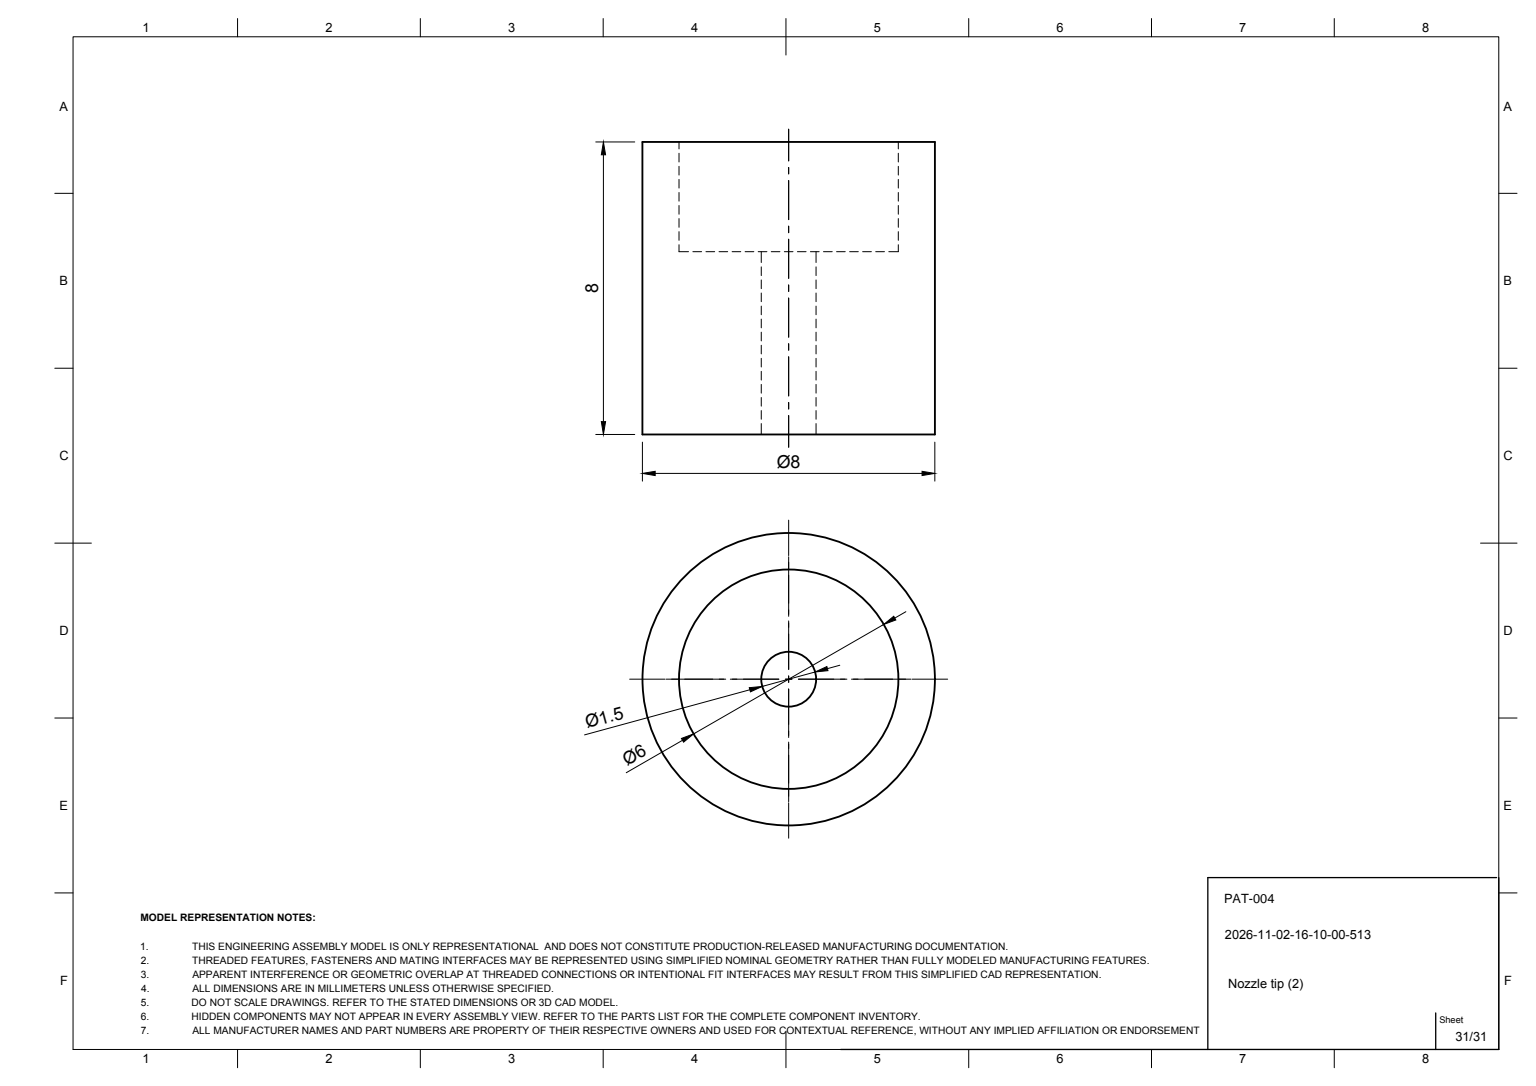
ISO-10303-21;
HEADER;
/* Generated by software containing ST-Developer
 * from STEP Tools, Inc. (www.steptools.com) 
 */

FILE_DESCRIPTION(
/* description */ ('Air blow-off nozzle station'),
/* implementation_level */ '2;1');

FILE_NAME(
/* name */ 'Nozzle tip (2).step',
/* time_stamp */ '2026-10-27T10:53:54-07:00',
/* author */ (''),
/* organization */ (''),
/* preprocessor_version */ 'ST-DEVELOPER v20.2',
/* originating_system */ 'Autodesk Translation Framework v15.17.0.0',
/* authorisation */ '');

FILE_SCHEMA (('AUTOMOTIVE_DESIGN { 1 0 10303 214 3 1 1 }'));
ENDSEC;

DATA;
#10=MECHANICAL_DESIGN_GEOMETRIC_PRESENTATION_REPRESENTATION('',(#259),#7897);
#209=SHAPE_REPRESENTATION_RELATIONSHIP('SRR','None',#8026,#234);
#234=ADVANCED_BREP_SHAPE_REPRESENTATION('',(#282),#7893);
#259=STYLED_ITEM('',(#8213),#282);
#282=MANIFOLD_SOLID_BREP('Body1',#4310);
#359=FACE_BOUND('',#1099,.T.);
#360=FACE_BOUND('',#1103,.T.);
#361=FACE_BOUND('',#1105,.T.);
#522=PLANE('',#5003);
#523=PLANE('',#5010);
#524=PLANE('',#5011);
#767=FACE_OUTER_BOUND('',#1097,.T.);
#768=FACE_OUTER_BOUND('',#1098,.T.);
#769=FACE_OUTER_BOUND('',#1100,.T.);
#770=FACE_OUTER_BOUND('',#1101,.T.);
#771=FACE_OUTER_BOUND('',#1102,.T.);
#772=FACE_OUTER_BOUND('',#1104,.T.);
#1097=EDGE_LOOP('',(#3857,#3858,#3859,#3860));
#1098=EDGE_LOOP('',(#3861));
#1099=EDGE_LOOP('',(#3862));
#1100=EDGE_LOOP('',(#3863,#3864,#3865,#3866));
#1101=EDGE_LOOP('',(#3867,#3868,#3869,#3870));
#1102=EDGE_LOOP('',(#3871));
#1103=EDGE_LOOP('',(#3872));
#1104=EDGE_LOOP('',(#3873));
#1105=EDGE_LOOP('',(#3874));
#1463=LINE('',#7703,#1817);
#1464=LINE('',#7710,#1818);
#1465=LINE('',#7716,#1819);
#1817=VECTOR('',#6223,0.3);
#1818=VECTOR('',#6232,0.0750000000000002);
#1819=VECTOR('',#6239,0.4);
#1985=CIRCLE('',#5001,0.3);
#1986=CIRCLE('',#5002,0.3);
#1987=CIRCLE('',#5004,0.0750000000000002);
#1988=CIRCLE('',#5006,0.0750000000000002);
#1989=CIRCLE('',#5008,0.4);
#1990=CIRCLE('',#5009,0.4);
#2332=VERTEX_POINT('',#7700);
#2333=VERTEX_POINT('',#7702);
#2334=VERTEX_POINT('',#7706);
#2335=VERTEX_POINT('',#7709);
#2336=VERTEX_POINT('',#7713);
#2337=VERTEX_POINT('',#7715);
#2846=EDGE_CURVE('',#2332,#2332,#1985,.T.);
#2847=EDGE_CURVE('',#2332,#2333,#1463,.T.);
#2848=EDGE_CURVE('',#2333,#2333,#1986,.T.);
#2849=EDGE_CURVE('',#2334,#2334,#1987,.T.);
#2850=EDGE_CURVE('',#2334,#2335,#1464,.T.);
#2851=EDGE_CURVE('',#2335,#2335,#1988,.T.);
#2852=EDGE_CURVE('',#2336,#2336,#1989,.T.);
#2853=EDGE_CURVE('',#2336,#2337,#1465,.T.);
#2854=EDGE_CURVE('',#2337,#2337,#1990,.T.);
#3857=ORIENTED_EDGE('',*,*,#2846,.F.);
#3858=ORIENTED_EDGE('',*,*,#2847,.T.);
#3859=ORIENTED_EDGE('',*,*,#2848,.F.);
#3860=ORIENTED_EDGE('',*,*,#2847,.F.);
#3861=ORIENTED_EDGE('',*,*,#2846,.T.);
#3862=ORIENTED_EDGE('',*,*,#2849,.F.);
#3863=ORIENTED_EDGE('',*,*,#2849,.T.);
#3864=ORIENTED_EDGE('',*,*,#2850,.T.);
#3865=ORIENTED_EDGE('',*,*,#2851,.T.);
#3866=ORIENTED_EDGE('',*,*,#2850,.F.);
#3867=ORIENTED_EDGE('',*,*,#2852,.F.);
#3868=ORIENTED_EDGE('',*,*,#2853,.T.);
#3869=ORIENTED_EDGE('',*,*,#2854,.T.);
#3870=ORIENTED_EDGE('',*,*,#2853,.F.);
#3871=ORIENTED_EDGE('',*,*,#2852,.T.);
#3872=ORIENTED_EDGE('',*,*,#2848,.T.);
#3873=ORIENTED_EDGE('',*,*,#2854,.F.);
#3874=ORIENTED_EDGE('',*,*,#2851,.F.);
#4019=CYLINDRICAL_SURFACE('',#5000,0.3);
#4020=CYLINDRICAL_SURFACE('',#5005,0.0750000000000002);
#4021=CYLINDRICAL_SURFACE('',#5007,0.4);
#4257=ADVANCED_FACE('',(#767),#4019,.F.);
#4258=ADVANCED_FACE('',(#768,#359),#522,.T.);
#4259=ADVANCED_FACE('',(#769),#4020,.F.);
#4260=ADVANCED_FACE('',(#770),#4021,.T.);
#4261=ADVANCED_FACE('',(#771,#360),#523,.T.);
#4262=ADVANCED_FACE('',(#772,#361),#524,.F.);
#4310=CLOSED_SHELL('',(#4257,#4258,#4259,#4260,#4261,#4262));
#4999=AXIS2_PLACEMENT_3D('',#7698,#6217,#6218);
#5000=AXIS2_PLACEMENT_3D('',#7699,#6219,#6220);
#5001=AXIS2_PLACEMENT_3D('',#7701,#6221,#6222);
#5002=AXIS2_PLACEMENT_3D('',#7704,#6224,#6225);
#5003=AXIS2_PLACEMENT_3D('',#7705,#6226,#6227);
#5004=AXIS2_PLACEMENT_3D('',#7707,#6228,#6229);
#5005=AXIS2_PLACEMENT_3D('',#7708,#6230,#6231);
#5006=AXIS2_PLACEMENT_3D('',#7711,#6233,#6234);
#5007=AXIS2_PLACEMENT_3D('',#7712,#6235,#6236);
#5008=AXIS2_PLACEMENT_3D('',#7714,#6237,#6238);
#5009=AXIS2_PLACEMENT_3D('',#7717,#6240,#6241);
#5010=AXIS2_PLACEMENT_3D('',#7718,#6242,#6243);
#5011=AXIS2_PLACEMENT_3D('',#7719,#6244,#6245);
#6217=DIRECTION('axis',(0.,0.,1.));
#6218=DIRECTION('refdir',(1.,0.,0.));
#6219=DIRECTION('center_axis',(0.,1.,0.));
#6220=DIRECTION('ref_axis',(1.,0.,0.));
#6221=DIRECTION('center_axis',(0.,1.,0.));
#6222=DIRECTION('ref_axis',(1.,0.,0.));
#6223=DIRECTION('',(0.,1.,0.));
#6224=DIRECTION('center_axis',(0.,-1.,0.));
#6225=DIRECTION('ref_axis',(1.,0.,0.));
#6226=DIRECTION('center_axis',(0.,1.,0.));
#6227=DIRECTION('ref_axis',(1.,0.,0.));
#6228=DIRECTION('center_axis',(0.,1.,0.));
#6229=DIRECTION('ref_axis',(1.,0.,0.));
#6230=DIRECTION('center_axis',(0.,1.,0.));
#6231=DIRECTION('ref_axis',(1.,0.,0.));
#6232=DIRECTION('',(0.,-1.,0.));
#6233=DIRECTION('center_axis',(0.,-1.,0.));
#6234=DIRECTION('ref_axis',(1.,0.,0.));
#6235=DIRECTION('center_axis',(0.,1.,0.));
#6236=DIRECTION('ref_axis',(1.,0.,0.));
#6237=DIRECTION('center_axis',(0.,1.,0.));
#6238=DIRECTION('ref_axis',(1.,0.,0.));
#6239=DIRECTION('',(0.,-1.,0.));
#6240=DIRECTION('center_axis',(0.,1.,0.));
#6241=DIRECTION('ref_axis',(1.,0.,0.));
#6242=DIRECTION('center_axis',(0.,1.,0.));
#6243=DIRECTION('ref_axis',(1.,0.,0.));
#6244=DIRECTION('center_axis',(0.,1.,0.));
#6245=DIRECTION('ref_axis',(1.,0.,0.));
#7698=CARTESIAN_POINT('',(0.,0.,0.));
#7699=CARTESIAN_POINT('Origin',(3.,-7.2,23.));
#7700=CARTESIAN_POINT('',(2.7,-7.2,23.));
#7701=CARTESIAN_POINT('Origin',(3.,-7.2,23.));
#7702=CARTESIAN_POINT('',(2.7,-6.9,23.));
#7703=CARTESIAN_POINT('',(2.7,-7.2,23.));
#7704=CARTESIAN_POINT('Origin',(3.,-6.9,23.));
#7705=CARTESIAN_POINT('Origin',(3.,-7.2,23.));
#7706=CARTESIAN_POINT('',(2.925,-7.2,23.));
#7707=CARTESIAN_POINT('Origin',(3.,-7.2,23.));
#7708=CARTESIAN_POINT('Origin',(3.,-7.7,23.));
#7709=CARTESIAN_POINT('',(2.925,-7.7,23.));
#7710=CARTESIAN_POINT('',(2.925,-7.7,23.));
#7711=CARTESIAN_POINT('Origin',(3.,-7.7,23.));
#7712=CARTESIAN_POINT('Origin',(3.,-7.7,23.));
#7713=CARTESIAN_POINT('',(2.6,-6.9,23.));
#7714=CARTESIAN_POINT('Origin',(3.,-6.9,23.));
#7715=CARTESIAN_POINT('',(2.6,-7.7,23.));
#7716=CARTESIAN_POINT('',(2.6,-7.7,23.));
#7717=CARTESIAN_POINT('Origin',(3.,-7.7,23.));
#7718=CARTESIAN_POINT('Origin',(3.,-6.9,23.));
#7719=CARTESIAN_POINT('Origin',(3.,-7.7,23.));
#7861=UNCERTAINTY_MEASURE_WITH_UNIT(LENGTH_MEASURE(0.001),#7898,
'DISTANCE_ACCURACY_VALUE',
'Maximum model space distance between geometric entities at asserted c
onnectivities');
#7865=UNCERTAINTY_MEASURE_WITH_UNIT(LENGTH_MEASURE(0.001),#7898,
'DISTANCE_ACCURACY_VALUE',
'Maximum model space distance between geometric entities at asserted c
onnectivities');
#7893=(
GEOMETRIC_REPRESENTATION_CONTEXT(3)
GLOBAL_UNCERTAINTY_ASSIGNED_CONTEXT((#7861))
GLOBAL_UNIT_ASSIGNED_CONTEXT((#7898,#7900,#7901))
REPRESENTATION_CONTEXT('','3D')
);
#7897=(
GEOMETRIC_REPRESENTATION_CONTEXT(3)
GLOBAL_UNCERTAINTY_ASSIGNED_CONTEXT((#7865))
GLOBAL_UNIT_ASSIGNED_CONTEXT((#7898,#7900,#7901))
REPRESENTATION_CONTEXT('','3D')
);
#7898=(
LENGTH_UNIT()
NAMED_UNIT(*)
SI_UNIT(.CENTI.,.METRE.)
);
#7900=(
NAMED_UNIT(*)
PLANE_ANGLE_UNIT()
SI_UNIT($,.RADIAN.)
);
#7901=(
NAMED_UNIT(*)
SI_UNIT($,.STERADIAN.)
SOLID_ANGLE_UNIT()
);
#7929=SHAPE_DEFINITION_REPRESENTATION(#7977,#8026);
#7977=PRODUCT_DEFINITION_SHAPE('',$,#8058);
#8026=SHAPE_REPRESENTATION('',(#4999),#7893);
#8030=PRODUCT_DEFINITION_CONTEXT('part definition',#8125,'design');
#8058=PRODUCT_DEFINITION('Nozzle tip (2)','Nozzle tip (2)',#8089,#8030);
#8089=PRODUCT_DEFINITION_FORMATION('',$,#8154);
#8125=APPLICATION_CONTEXT(
'Core Data for Automotive Mechanical Design Process');
#8126=PRODUCT_CONTEXT('part definition',#8125,'mechanical');
#8154=PRODUCT('Nozzle tip (2)','Nozzle tip (2)','Nozzle tip (2)',(#8126));
#8207=COLOUR_RGB('Sky Blue',0.24,0.69,0.87);
#8208=FILL_AREA_STYLE_COLOUR('',#8207);
#8209=FILL_AREA_STYLE('',(#8208));
#8210=SURFACE_STYLE_FILL_AREA(#8209);
#8211=SURFACE_SIDE_STYLE('',(#8210));
#8212=SURFACE_STYLE_USAGE(.BOTH.,#8211);
#8213=PRESENTATION_STYLE_ASSIGNMENT((#8212));
ENDSEC;
END-ISO-10303-21;
